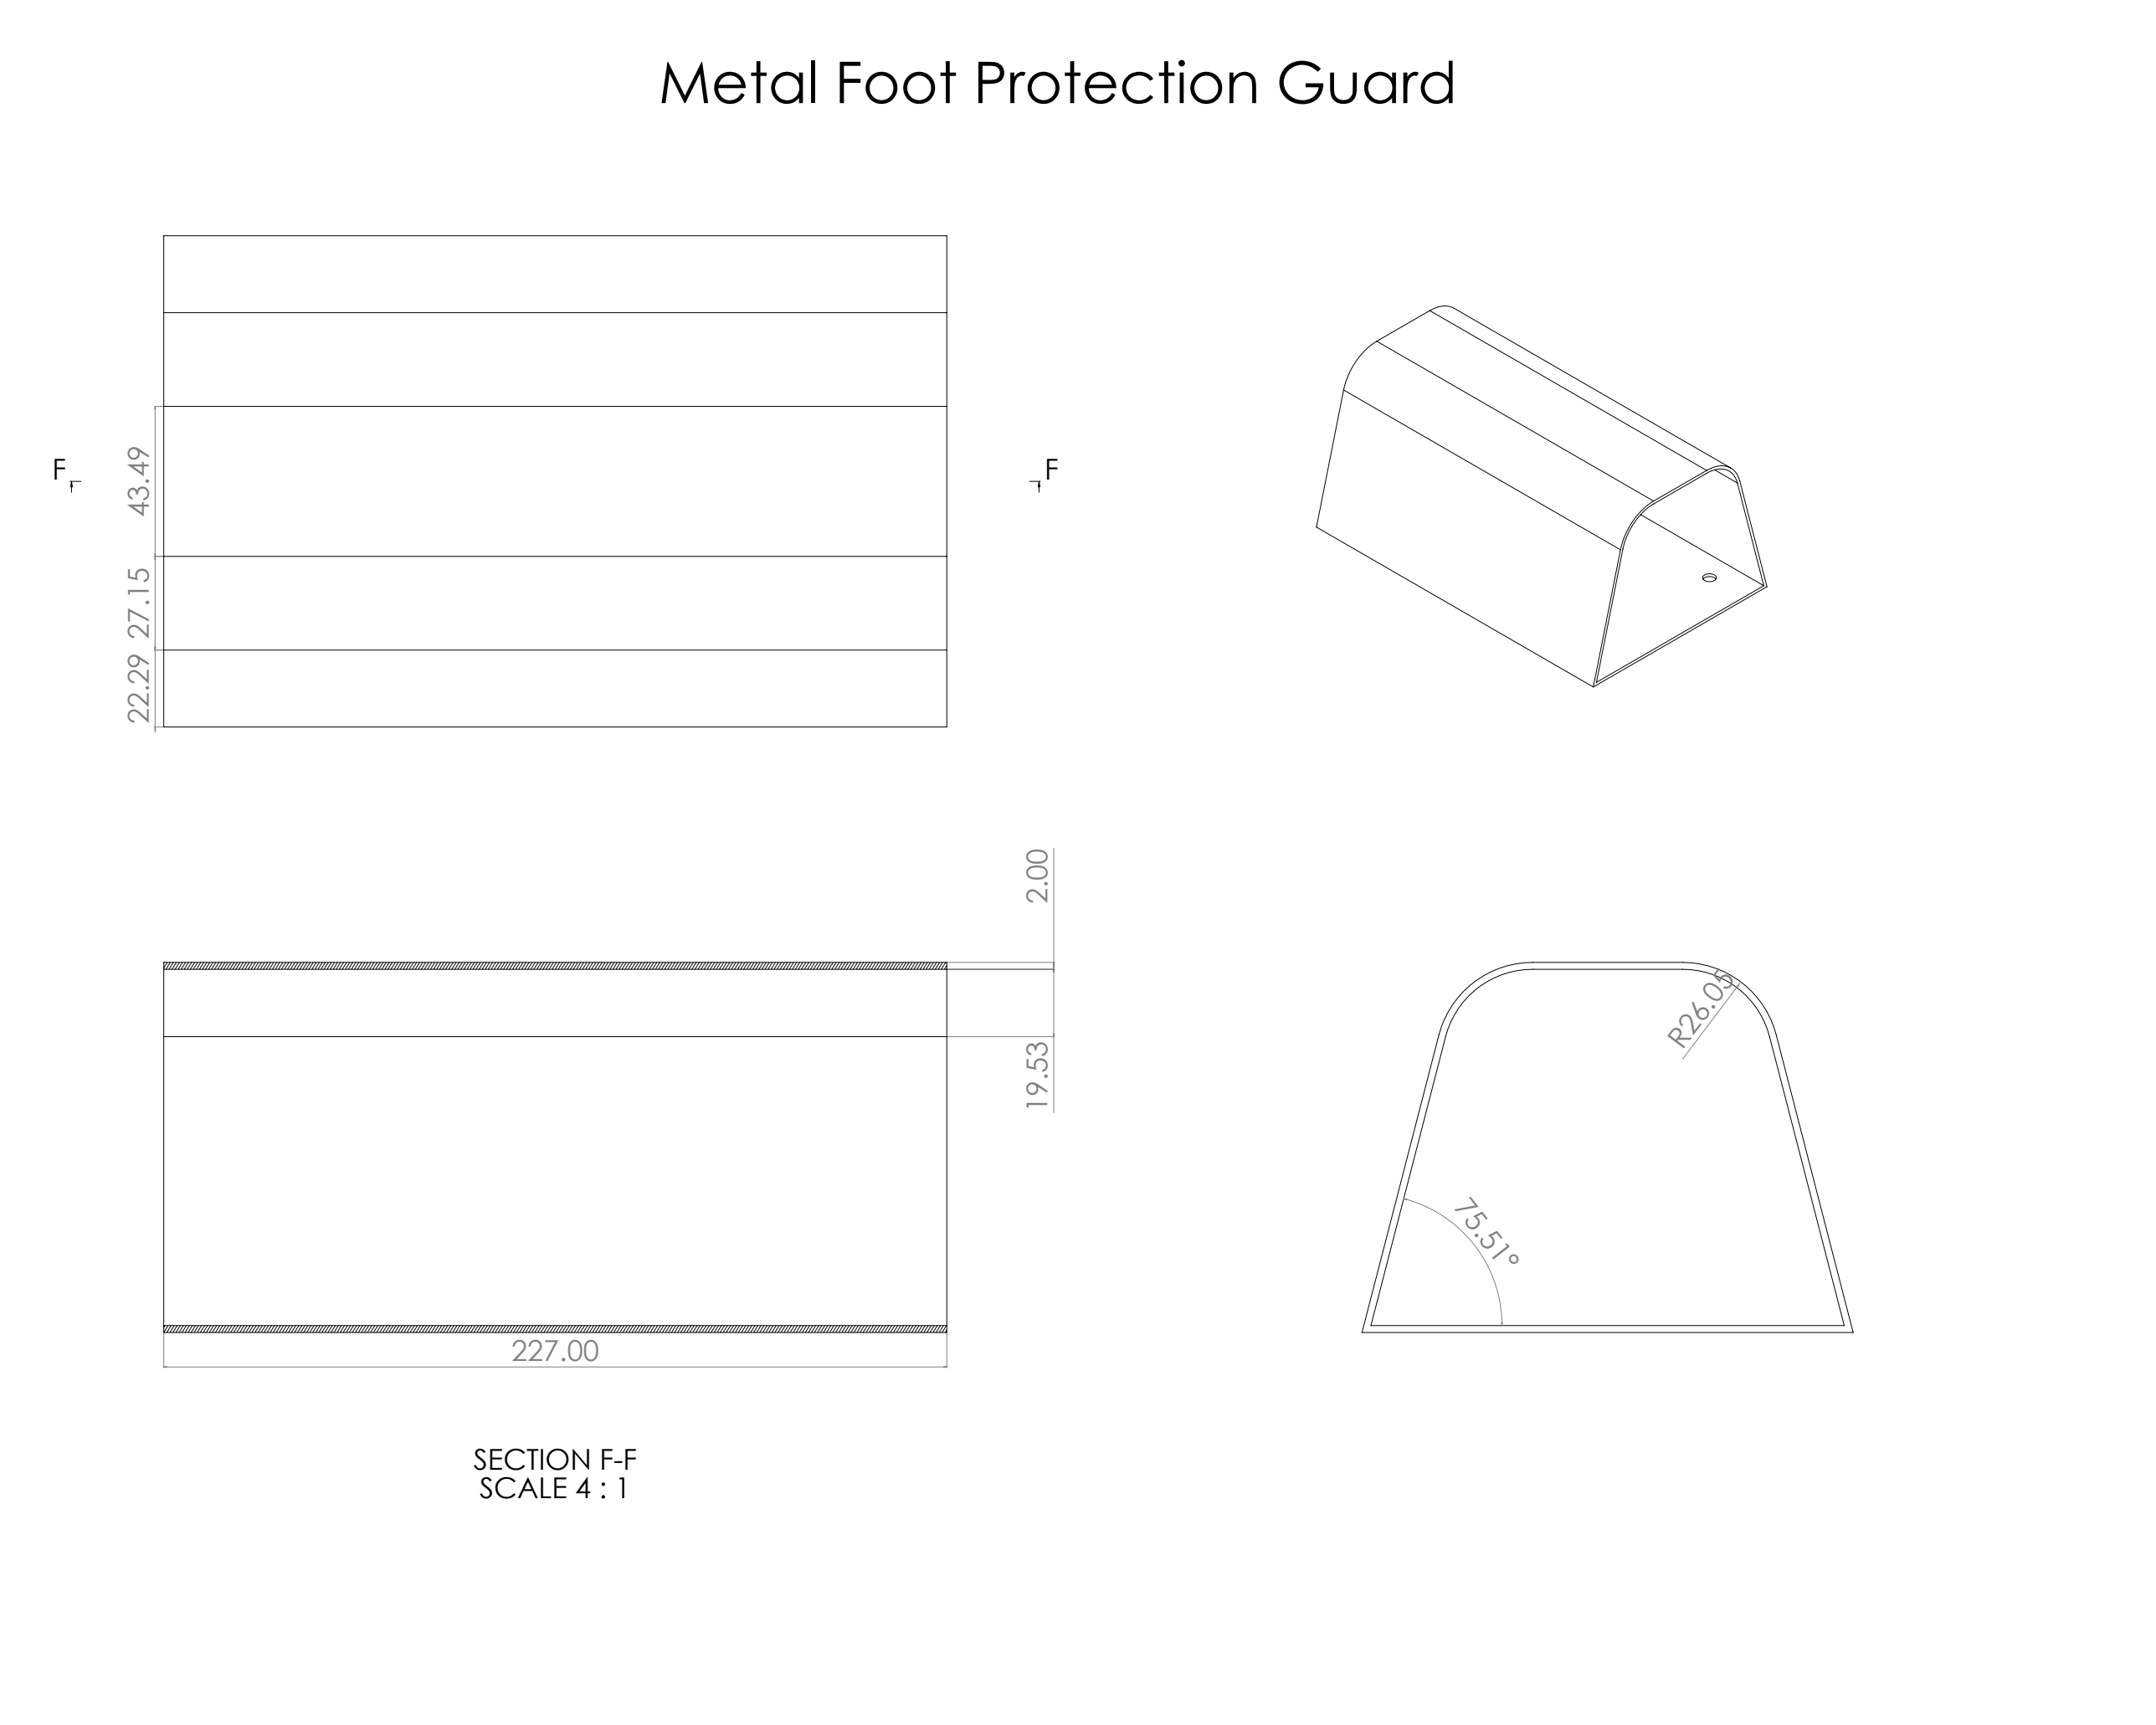
ISO-10303-21;
HEADER;
FILE_DESCRIPTION (('STEP AP214'),
    '1' );
FILE_NAME ('Metal Foot Protection Guard.step',
    '2026-10-25T20:52:49',
    ( '' ),
    ( '' ),
    'SwSTEP 2.0',
    'SolidWorks 2025',
    '' );
FILE_SCHEMA (( 'AUTOMOTIVE_DESIGN' ));
ENDSEC;

DATA;
#6=DIRECTION ( 'NONE',  ( 0.000000000000000000, 1.000000000000000000, 0.000000000000000000 ) ) ;
#417=ORIENTED_EDGE ( 'NONE', *, *, #24378, .F. ) ;
#442=ORIENTED_EDGE ( 'NONE', *, *, #84617, .T. ) ;
#778=VECTOR ( 'NONE', #36386, 1000.000000000000000 ) ;
#1124=ORIENTED_EDGE ( 'NONE', *, *, #88943, .T. ) ;
#1238=PLANE ( 'NONE',  #55318 ) ;
#1278=CARTESIAN_POINT ( 'NONE',  ( -113.5000000000000568, -218.8335761803644743, -447.4016117689005796 ) ) ;
#1316=LINE ( 'NONE', #58628, #74329 ) ;
#1432=CYLINDRICAL_SURFACE ( 'NONE', #55768, 26.04691768583017364 ) ;
#1539=DIRECTION ( 'NONE',  ( -1.000000000000000000, -0.000000000000000000, -0.000000000000000000 ) ) ;
#1792=LINE ( 'NONE', #80865, #778 ) ;
#1878=ORIENTED_EDGE ( 'NONE', *, *, #16109, .T. ) ;
#1900=DIRECTION ( 'NONE',  ( -1.000000000000000000, -0.000000000000000000, -0.000000000000000000 ) ) ;
#1936=ORIENTED_EDGE ( 'NONE', *, *, #63556, .T. ) ;
#1958=PRODUCT ( 'Metal Foot Protection Guard', 'Metal Foot Protection Guard', '', ( #38817 ) ) ;
#2011=AXIS2_PLACEMENT_3D ( 'NONE', #16154, #66807, #89023 ) ;
#2249=LINE ( 'NONE', #31133, #23268 ) ;
#2276=VERTEX_POINT ( 'NONE', #93668 ) ;
#2307=ORIENTED_EDGE ( 'NONE', *, *, #76975, .F. ) ;
#2323=VECTOR ( 'NONE', #62128, 1000.000000000000114 ) ;
#2326=DIRECTION ( 'NONE',  ( 0.000000000000000000, 1.000000000000000000, 0.000000000000000000 ) ) ;
#2997=CARTESIAN_POINT ( 'NONE',  ( -83.63170945779077670, -296.0521521680024080, -417.1172536214571096 ) ) ;
#3014=DIRECTION ( 'NONE',  ( 0.000000000000000000, 0.000000000000000000, 1.000000000000000000 ) ) ;
#3055=CARTESIAN_POINT ( 'NONE',  ( 113.5000000000000568, -218.8335761803644743, -490.8867980474134356 ) ) ;
#3161=ORIENTED_EDGE ( 'NONE', *, *, #12809, .F. ) ;
#3235=EDGE_CURVE ( 'NONE', #62642, #12065, #46260, .T. ) ;
#3595=AXIS2_PLACEMENT_3D ( 'NONE', #45296, #24471, #37283 ) ;
#3602=LINE ( 'NONE', #11632, #79019 ) ;
#3637=AXIS2_PLACEMENT_3D ( 'NONE', #49476, #63245, #84503 ) ;
#3779=ADVANCED_FACE ( 'NONE', ( #26838 ), #85054, .T. ) ;
#4574=UNCERTAINTY_MEASURE_WITH_UNIT (LENGTH_MEASURE( 1.000000000000000082E-05 ), #34987, 'distance_accuracy_value', 'NONE');
#4833=EDGE_CURVE ( 'NONE', #43507, #93231, #73286, .T. ) ;
#4839=ORIENTED_EDGE ( 'NONE', *, *, #80738, .T. ) ;
#4990=AXIS2_PLACEMENT_3D ( 'NONE', #56009, #66271, #51112 ) ;
#5017=CIRCLE ( 'NONE', #18666, 4.000000000000003553 ) ;
#5158=ORIENTED_EDGE ( 'NONE', *, *, #48217, .F. ) ;
#5173=ORIENTED_EDGE ( 'NONE', *, *, #11459, .F. ) ;
#5210=ORIENTED_EDGE ( 'NONE', *, *, #44156, .F. ) ;
#5394=ORIENTED_EDGE ( 'NONE', *, *, #33276, .T. ) ;
#5925=DIRECTION ( 'NONE',  ( 0.000000000000000000, 0.000000000000000000, 1.000000000000000000 ) ) ;
#6052=PLANE ( 'NONE',  #74600 ) ;
#6401=DIRECTION ( 'NONE',  ( 0.000000000000000000, -0.2502735790305607444, 0.9681751575201843485 ) ) ;
#6492=VECTOR ( 'NONE', #33731, 1000.000000000000000 ) ;
#6796=ORIENTED_EDGE ( 'NONE', *, *, #27340, .T. ) ;
#6987=FACE_BOUND ( 'NONE', #78000, .T. ) ;
#7172=( LENGTH_UNIT ( ) NAMED_UNIT ( * ) SI_UNIT ( .MILLI., .METRE. ) );
#7304=EDGE_LOOP ( 'NONE', ( #59580, #39641, #11949, #25899 ) ) ;
#7427=VECTOR ( 'NONE', #91516, 1000.000000000000000 ) ;
#7537=CARTESIAN_POINT ( 'NONE',  ( 113.5000000000000568, -296.0521521680024080, -400.5374811273811702 ) ) ;
#7762=PRODUCT_DEFINITION_CONTEXT ( 'detailed design', #78364, 'design' ) ;
#8035=VECTOR ( 'NONE', #18647, 1000.000000000000000 ) ;
#8052=AXIS2_PLACEMENT_3D ( 'NONE', #67191, #2326, #31206 ) ;
#8263=VECTOR ( 'NONE', #42060, 1000.000000000000000 ) ;
#8490=CARTESIAN_POINT ( 'NONE',  ( 113.5000000000000568, -296.0521521680024080, -537.7509286889328450 ) ) ;
#8572=ADVANCED_FACE ( 'NONE', ( #49622 ), #42507, .F. ) ;
#8832=VECTOR ( 'NONE', #60146, 1000.000000000000000 ) ;
#9134=DIRECTION ( 'NONE',  ( 0.000000000000000000, 0.000000000000000000, 1.000000000000000000 ) ) ;
#9174=CARTESIAN_POINT ( 'NONE',  ( -83.63170945779074827, -298.0521521680024080, -525.1711561948568487 ) ) ;
#9287=DIRECTION ( 'NONE',  ( 0.000000000000000000, 0.000000000000000000, 1.000000000000000000 ) ) ;
#9340=CARTESIAN_POINT ( 'NONE',  ( -113.5000000000000568, -298.0521521680024080, -397.9547385950631337 ) ) ;
#9353=EDGE_CURVE ( 'NONE', #42812, #91222, #48447, .T. ) ;
#9407=LINE ( 'NONE', #9886, #56602 ) ;
#9526=CIRCLE ( 'NONE', #18677, 4.000000000000003553 ) ;
#9540=ORIENTED_EDGE ( 'NONE', *, *, #63681, .T. ) ;
#9616=VERTEX_POINT ( 'NONE', #11064 ) ;
#9664=VECTOR ( 'NONE', #74863, 1000.000000000000000 ) ;
#9758=LINE ( 'NONE', #89272, #23223 ) ;
#9886=CARTESIAN_POINT ( 'NONE',  ( -83.63170945779074827, -373.0521521680024648, -517.1711561948568487 ) ) ;
#10053=CARTESIAN_POINT ( 'NONE',  ( -113.5000000000000568, -296.0521521680024080, -400.5374811273811702 ) ) ;
#10064=DIRECTION ( 'NONE',  ( 0.000000000000000000, 0.000000000000000000, -1.000000000000000000 ) ) ;
#10078=ORIENTED_EDGE ( 'NONE', *, *, #83711, .T. ) ;
#10254=VERTEX_POINT ( 'NONE', #23518 ) ;
#10301=DIRECTION ( 'NONE',  ( -1.000000000000000000, -0.000000000000000000, -0.000000000000000000 ) ) ;
#10703=CARTESIAN_POINT ( 'NONE',  ( -113.5000000000000568, -212.3147208684173677, -516.1047766808072765 ) ) ;
#10768=DIRECTION ( 'NONE',  ( 0.000000000000000000, 1.000000000000000000, -0.000000000000000000 ) ) ;
#11004=CARTESIAN_POINT ( 'NONE',  ( -113.5000000000000568, -192.7866584945343504, -447.4016117689005796 ) ) ;
#11062=ORIENTED_EDGE ( 'NONE', *, *, #17386, .T. ) ;
#11064=CARTESIAN_POINT ( 'NONE',  ( -83.63170945779077670, -296.0521521680024080, -421.1172536214571096 ) ) ;
#11141=VECTOR ( 'NONE', #68705, 1000.000000000000000 ) ;
#11159=CIRCLE ( 'NONE', #3595, 4.000000000000003553 ) ;
#11217=VECTOR ( 'NONE', #42131, 1000.000000000000000 ) ;
#11220=AXIS2_PLACEMENT_3D ( 'NONE', #68307, #26618, #10064 ) ;
#11228=CIRCLE ( 'NONE', #12737, 4.000000000000003553 ) ;
#11384=CARTESIAN_POINT ( 'NONE',  ( 85.55100297371598117, -373.0521521680024648, -417.1172536214571096 ) ) ;
#11459=EDGE_CURVE ( 'NONE', #56922, #42812, #78843, .T. ) ;
#11572=ORIENTED_EDGE ( 'NONE', *, *, #57340, .F. ) ;
#11597=ADVANCED_FACE ( 'NONE', ( #34821 ), #92559, .F. ) ;
#11632=CARTESIAN_POINT ( 'NONE',  ( 113.5000000000000568, -192.7866584945343504, -490.8867980474134356 ) ) ;
#11690=LINE ( 'NONE', #31611, #47780 ) ;
#11793=VERTEX_POINT ( 'NONE', #9174 ) ;
#11949=ORIENTED_EDGE ( 'NONE', *, *, #24378, .T. ) ;
#11985=FACE_OUTER_BOUND ( 'NONE', #85658, .T. ) ;
#12065=VERTEX_POINT ( 'NONE', #81159 ) ;
#12119=DIRECTION ( 'NONE',  ( 0.000000000000000000, 0.000000000000000000, 1.000000000000000000 ) ) ;
#12292=AXIS2_PLACEMENT_3D ( 'NONE', #39594, #90715, #47174 ) ;
#12596=DIRECTION ( 'NONE',  ( 0.000000000000000000, 0.000000000000000000, 1.000000000000000000 ) ) ;
#12668=VECTOR ( 'NONE', #72103, 1000.000000000000000 ) ;
#12724=AXIS2_PLACEMENT_3D ( 'NONE', #43548, #6, #35985 ) ;
#12737=AXIS2_PLACEMENT_3D ( 'NONE', #90881, #26997, #70096 ) ;
#12809=EDGE_CURVE ( 'NONE', #47975, #62368, #77199, .T. ) ;
#13122=DIRECTION ( 'NONE',  ( 0.000000000000000000, 0.000000000000000000, 1.000000000000000000 ) ) ;
#13127=ORIENTED_EDGE ( 'NONE', *, *, #73397, .F. ) ;
#13224=LINE ( 'NONE', #63892, #8263 ) ;
#13625=EDGE_CURVE ( 'NONE', #81684, #49342, #44460, .T. ) ;
#13690=CARTESIAN_POINT ( 'NONE',  ( -113.5000000000000568, -296.0521521680024080, -537.7509286889328450 ) ) ;
#13868=EDGE_CURVE ( 'NONE', #10254, #49342, #9407, .T. ) ;
#14078=ORIENTED_EDGE ( 'NONE', *, *, #37019, .F. ) ;
#14096=FACE_OUTER_BOUND ( 'NONE', #76110, .T. ) ;
#14616=FACE_BOUND ( 'NONE', #27456, .T. ) ;
#14990=DIRECTION ( 'NONE',  ( -1.000000000000000000, -0.000000000000000000, -0.000000000000000000 ) ) ;
#15544=VECTOR ( 'NONE', #14990, 1000.000000000000000 ) ;
#15625=EDGE_LOOP ( 'NONE', ( #53579, #46500, #71098, #20534 ) ) ;
#15643=FACE_OUTER_BOUND ( 'NONE', #7304, .T. ) ;
#15682=VECTOR ( 'NONE', #78384, 1000.000000000000000 ) ;
#15729=CARTESIAN_POINT ( 'NONE',  ( 113.5000000000000568, -218.8335761803644743, -490.8867980474134356 ) ) ;
#16109=EDGE_CURVE ( 'NONE', #36642, #59451, #59215, .T. ) ;
#16152=ORIENTED_EDGE ( 'NONE', *, *, #87773, .F. ) ;
#16154=CARTESIAN_POINT ( 'NONE',  ( 113.5000000000000568, -298.0521521680024080, -397.9547385950631337 ) ) ;
#16280=DIRECTION ( 'NONE',  ( 0.000000000000000000, 1.000000000000000000, -0.000000000000000000 ) ) ;
#16610=VERTEX_POINT ( 'NONE', #17359 ) ;
#16751=CARTESIAN_POINT ( 'NONE',  ( 85.55100297371598117, -298.0521521680024080, -413.1172536214571096 ) ) ;
#17028=EDGE_CURVE ( 'NONE', #11793, #10254, #78948, .T. ) ;
#17038=PLANE ( 'NONE',  #56694 ) ;
#17200=CYLINDRICAL_SURFACE ( 'NONE', #59412, 4.000000000000003553 ) ;
#17359=CARTESIAN_POINT ( 'NONE',  ( 85.55100297371609486, -296.0521521680024080, -517.1711561948568487 ) ) ;
#17386=EDGE_CURVE ( 'NONE', #83022, #62368, #77460, .T. ) ;
#17968=DIRECTION ( 'NONE',  ( 0.000000000000000000, -0.9681751575201845705, -0.2502735790305594121 ) ) ;
#18379=AXIS2_PLACEMENT_3D ( 'NONE', #1278, #36796, #9287 ) ;
#18420=ORIENTED_EDGE ( 'NONE', *, *, #41482, .F. ) ;
#18451=EDGE_LOOP ( 'NONE', ( #81543, #43240, #57627, #38795 ) ) ;
#18490=CARTESIAN_POINT ( 'NONE',  ( 85.55100297371598117, -373.0521521680024648, -421.1172536214571096 ) ) ;
#18518=ORIENTED_EDGE ( 'NONE', *, *, #62083, .T. ) ;
#18585=ORIENTED_EDGE ( 'NONE', *, *, #17028, .F. ) ;
#18647=DIRECTION ( 'NONE',  ( 0.000000000000000000, 0.000000000000000000, -1.000000000000000000 ) ) ;
#18666=AXIS2_PLACEMENT_3D ( 'NONE', #60916, #53801, #89762 ) ;
#18677=AXIS2_PLACEMENT_3D ( 'NONE', #58278, #92351, #27995 ) ;
#18940=AXIS2_PLACEMENT_3D ( 'NONE', #90959, #40773, #33703 ) ;
#18980=LINE ( 'NONE', #83344, #11141 ) ;
#19066=LINE ( 'NONE', #54562, #47269 ) ;
#19232=PRODUCT_DEFINITION ( 'UNKNOWN', '', #50708, #7762 ) ;
#19258=ORIENTED_EDGE ( 'NONE', *, *, #88840, .T. ) ;
#19434=CARTESIAN_POINT ( 'NONE',  ( 113.5000000000000568, -190.7866584945343220, -490.8867980474134356 ) ) ;
#19749=LINE ( 'NONE', #49566, #47581 ) ;
#19761=EDGE_LOOP ( 'NONE', ( #31495, #72178, #26521, #82940 ) ) ;
#19828=ORIENTED_EDGE ( 'NONE', *, *, #17386, .F. ) ;
#19877=ORIENTED_EDGE ( 'NONE', *, *, #47034, .T. ) ;
#20150=EDGE_CURVE ( 'NONE', #62642, #36954, #86465, .T. ) ;
#20278=CIRCLE ( 'NONE', #3637, 4.000000000000003553 ) ;
#20299=ORIENTED_EDGE ( 'NONE', *, *, #63681, .F. ) ;
#20534=ORIENTED_EDGE ( 'NONE', *, *, #20150, .T. ) ;
#20637=DIRECTION ( 'NONE',  ( 0.000000000000000000, 0.000000000000000000, 1.000000000000000000 ) ) ;
#21150=ORIENTED_EDGE ( 'NONE', *, *, #37532, .F. ) ;
#21204=ADVANCED_FACE ( 'NONE', ( #39998 ), #34334, .F. ) ;
#21313=CARTESIAN_POINT ( 'NONE',  ( 113.5000000000000568, -211.8141737103562434, -420.2472828204663529 ) ) ;
#21449=ORIENTED_EDGE ( 'NONE', *, *, #40622, .F. ) ;
#21618=CIRCLE ( 'NONE', #66969, 26.04691768583017364 ) ;
#22565=DIRECTION ( 'NONE',  ( 0.000000000000000000, 0.9681751575201842375, 0.2502735790305606889 ) ) ;
#22793=EDGE_CURVE ( 'NONE', #29874, #9616, #86552, .T. ) ;
#22928=LINE ( 'NONE', #23410, #36160 ) ;
#23184=VECTOR ( 'NONE', #47355, 1000.000000000000000 ) ;
#23194=CARTESIAN_POINT ( 'NONE',  ( -83.63170945779074827, -296.0521521680024080, -525.1711561948568487 ) ) ;
#23223=VECTOR ( 'NONE', #22565, 1000.000000000000114 ) ;
#23268=VECTOR ( 'NONE', #60019, 1000.000000000000114 ) ;
#23410=CARTESIAN_POINT ( 'NONE',  ( 113.5000000000000568, -298.0521521680024080, -397.9547385950631337 ) ) ;
#23518=CARTESIAN_POINT ( 'NONE',  ( -83.63170945779074827, -298.0521521680024080, -517.1711561948568487 ) ) ;
#24130=FACE_BOUND ( 'NONE', #61458, .T. ) ;
#24202=CARTESIAN_POINT ( 'NONE',  ( 113.5000000000000568, -192.7866584945343504, -447.4016117689005796 ) ) ;
#24218=ORIENTED_EDGE ( 'NONE', *, *, #20150, .F. ) ;
#24378=EDGE_CURVE ( 'NONE', #59329, #45702, #21618, .T. ) ;
#24471=DIRECTION ( 'NONE',  ( 0.000000000000000000, 1.000000000000000000, -0.000000000000000000 ) ) ;
#24482=CYLINDRICAL_SURFACE ( 'NONE', #12292, 4.000000000000003553 ) ;
#24501=ADVANCED_FACE ( 'NONE', ( #49483 ), #42361, .T. ) ;
#24656=CARTESIAN_POINT ( 'NONE',  ( 113.5000000000000568, -190.7866584945343504, -447.4016117689005796 ) ) ;
#24719=AXIS2_PLACEMENT_3D ( 'NONE', #52941, #58675, #80428 ) ;
#24795=AXIS2_PLACEMENT_3D ( 'NONE', #83095, #46641, #61365 ) ;
#24966=VERTEX_POINT ( 'NONE', #16751 ) ;
#24977=DIRECTION ( 'NONE',  ( 0.000000000000000000, 0.9681751575201845705, 0.2502735790305594676 ) ) ;
#25097=EDGE_CURVE ( 'NONE', #36396, #62468, #29192, .T. ) ;
#25137=DIRECTION ( 'NONE',  ( -1.000000000000000000, -0.000000000000000000, -0.000000000000000000 ) ) ;
#25427=CARTESIAN_POINT ( 'NONE',  ( -83.63170945779077670, -298.0521521680024080, -421.1172536214571096 ) ) ;
#25499=CARTESIAN_POINT ( 'NONE',  ( -83.63170945779077670, -298.0521521680024080, -417.1172536214571096 ) ) ;
#25663=VECTOR ( 'NONE', #69750, 1000.000000000000000 ) ;
#25825=CARTESIAN_POINT ( 'NONE',  ( 85.55100297371609486, -373.0521521680024648, -517.1711561948568487 ) ) ;
#25899=ORIENTED_EDGE ( 'NONE', *, *, #27474, .T. ) ;
#25906=ADVANCED_FACE ( 'NONE', ( #63142 ), #92435, .F. ) ;
#25988=CARTESIAN_POINT ( 'NONE',  ( -113.5000000000000568, -211.8141737103562434, -420.2472828204663529 ) ) ;
#26374=AXIS2_PLACEMENT_3D ( 'NONE', #11384, #55885, #77662 ) ;
#26406=CARTESIAN_POINT ( 'NONE',  ( -83.63170945779077670, -296.0521521680024080, -413.1172536214571096 ) ) ;
#26521=ORIENTED_EDGE ( 'NONE', *, *, #92612, .F. ) ;
#26576=STYLED_ITEM('',(#93745),#91220);
#26618=DIRECTION ( 'NONE',  ( 1.000000000000000000, 0.000000000000000000, 0.000000000000000000 ) ) ;
#26725=VERTEX_POINT ( 'NONE', #31215 ) ;
#26753=ORIENTED_EDGE ( 'NONE', *, *, #54874, .F. ) ;
#26784=LINE ( 'NONE', #69395, #69956 ) ;
#26790=DIRECTION ( 'NONE',  ( 0.000000000000000000, 0.000000000000000000, -1.000000000000000000 ) ) ;
#26838=FACE_OUTER_BOUND ( 'NONE', #29382, .T. ) ;
#26936=DIRECTION ( 'NONE',  ( -0.000000000000000000, 1.000000000000000000, 0.000000000000000000 ) ) ;
#26993=EDGE_CURVE ( 'NONE', #62368, #42343, #66156, .T. ) ;
#26997=DIRECTION ( 'NONE',  ( -0.000000000000000000, 1.000000000000000000, 0.000000000000000000 ) ) ;
#27340=EDGE_CURVE ( 'NONE', #86290, #16610, #41184, .T. ) ;
#27456=EDGE_LOOP ( 'NONE', ( #13127, #57449 ) ) ;
#27474=EDGE_CURVE ( 'NONE', #45702, #59451, #26784, .T. ) ;
#27503=EDGE_CURVE ( 'NONE', #32344, #93231, #3602, .T. ) ;
#27715=DIRECTION ( 'NONE',  ( 1.000000000000000000, 0.000000000000000000, -0.000000000000000000 ) ) ;
#27811=AXIS2_PLACEMENT_3D ( 'NONE', #92152, #71340, #13122 ) ;
#27995=DIRECTION ( 'NONE',  ( 0.000000000000000000, 0.000000000000000000, 1.000000000000000000 ) ) ;
#28110=ORIENTED_EDGE ( 'NONE', *, *, #46184, .T. ) ;
#28339=VERTEX_POINT ( 'NONE', #72116 ) ;
#28547=DIRECTION ( 'NONE',  ( 1.000000000000000000, 0.000000000000000000, 0.000000000000000000 ) ) ;
#28573=ORIENTED_EDGE ( 'NONE', *, *, #84617, .F. ) ;
#28694=ADVANCED_FACE ( 'NONE', ( #38416 ), #89059, .T. ) ;
#28804=CIRCLE ( 'NONE', #43914, 4.000000000000003553 ) ;
#28860=ORIENTED_EDGE ( 'NONE', *, *, #92612, .T. ) ;
#29034=LINE ( 'NONE', #65051, #79325 ) ;
#29126=VECTOR ( 'NONE', #88842, 1000.000000000000000 ) ;
#29188=CARTESIAN_POINT ( 'NONE',  ( -113.5000000000000568, -218.8335761803644743, -447.4016117689005796 ) ) ;
#29192=CIRCLE ( 'NONE', #42837, 4.000000000000003553 ) ;
#29382=EDGE_LOOP ( 'NONE', ( #47639, #21150, #5210, #41236 ) ) ;
#29514=CLOSED_SHELL ( 'NONE', ( #63024, #58384, #8572, #25906, #86201, #90366, #64306, #71705, #86978, #28694, #11597, #3779, #45814, #65404, #57136, #24501, #56322, #67787, #21204, #57559, #74931, #33563 ) ) ;
#29531=ORIENTED_EDGE ( 'NONE', *, *, #72303, .F. ) ;
#29874=VERTEX_POINT ( 'NONE', #26406 ) ;
#30154=DIRECTION ( 'NONE',  ( -0.000000000000000000, -0.000000000000000000, 1.000000000000000000 ) ) ;
#30209=CARTESIAN_POINT ( 'NONE',  ( -83.63170945779077670, -373.0521521680024648, -421.1172536214571096 ) ) ;
#30870=DIRECTION ( 'NONE',  ( -1.000000000000000000, -0.000000000000000000, -0.000000000000000000 ) ) ;
#30965=DIRECTION ( 'NONE',  ( 0.000000000000000000, 0.000000000000000000, -1.000000000000000000 ) ) ;
#31133=CARTESIAN_POINT ( 'NONE',  ( 113.5000000000000568, -296.0521521680024080, -400.5374811273811702 ) ) ;
#31206=DIRECTION ( 'NONE',  ( 0.000000000000000000, 0.000000000000000000, 1.000000000000000000 ) ) ;
#31215=CARTESIAN_POINT ( 'NONE',  ( -113.5000000000000568, -298.0521521680024080, -397.9547385950631337 ) ) ;
#31299=FACE_OUTER_BOUND ( 'NONE', #48421, .T. ) ;
#31495=ORIENTED_EDGE ( 'NONE', *, *, #26993, .T. ) ;
#31611=CARTESIAN_POINT ( 'NONE',  ( 85.55100297371598117, -373.0521521680024648, -413.1172536214571096 ) ) ;
#32008=CARTESIAN_POINT ( 'NONE',  ( -113.5000000000000568, -190.7866584945343504, -447.4016117689005796 ) ) ;
#32177=FACE_OUTER_BOUND ( 'NONE', #62147, .T. ) ;
#32191=VERTEX_POINT ( 'NONE', #48875 ) ;
#32344=VERTEX_POINT ( 'NONE', #73466 ) ;
#32571=DIRECTION ( 'NONE',  ( 1.000000000000000000, 0.000000000000000000, -0.000000000000000000 ) ) ;
#32846=EDGE_CURVE ( 'NONE', #33034, #42343, #75779, .T. ) ;
#33034=VERTEX_POINT ( 'NONE', #52591 ) ;
#33131=ORIENTED_EDGE ( 'NONE', *, *, #88943, .F. ) ;
#33276=EDGE_CURVE ( 'NONE', #24966, #2276, #11228, .T. ) ;
#33562=PLANE ( 'NONE',  #73301 ) ;
#33563=ADVANCED_FACE ( 'NONE', ( #33622 ), #77187, .F. ) ;
#33622=FACE_OUTER_BOUND ( 'NONE', #60401, .T. ) ;
#33703=DIRECTION ( 'NONE',  ( 1.000000000000000000, 0.000000000000000000, 0.000000000000000000 ) ) ;
#33731=DIRECTION ( 'NONE',  ( -0.000000000000000000, -0.000000000000000000, 1.000000000000000000 ) ) ;
#33765=LINE ( 'NONE', #40831, #25663 ) ;
#33970=CARTESIAN_POINT ( 'NONE',  ( 85.55100297371598117, -296.0521521680024080, -421.1172536214571096 ) ) ;
#34334=CYLINDRICAL_SURFACE ( 'NONE', #42697, 4.000000000000003553 ) ;
#34351=EDGE_CURVE ( 'NONE', #62468, #36396, #38245, .T. ) ;
#34433=EDGE_LOOP ( 'NONE', ( #5394, #4839 ) ) ;
#34821=FACE_OUTER_BOUND ( 'NONE', #19761, .T. ) ;
#34974=ORIENTED_EDGE ( 'NONE', *, *, #93458, .F. ) ;
#34975=FACE_BOUND ( 'NONE', #60847, .T. ) ;
#34987=( LENGTH_UNIT ( ) NAMED_UNIT ( * ) SI_UNIT ( .MILLI., .METRE. ) );
#35165=CARTESIAN_POINT ( 'NONE',  ( -83.63170945779077670, -373.0521521680024648, -417.1172536214571096 ) ) ;
#35273=DIRECTION ( 'NONE',  ( 0.000000000000000000, -0.9681751575201842375, -0.2502735790305606889 ) ) ;
#35461=ORIENTED_EDGE ( 'NONE', *, *, #65933, .F. ) ;
#35632=EDGE_CURVE ( 'NONE', #28339, #43507, #57427, .T. ) ;
#35763=CARTESIAN_POINT ( 'NONE',  ( 113.5000000000000568, -296.0521521680024080, -400.5374811273811702 ) ) ;
#35912=CARTESIAN_POINT ( 'NONE',  ( 113.5000000000000568, -296.0521521680024080, -400.5374811273811702 ) ) ;
#35985=DIRECTION ( 'NONE',  ( 0.000000000000000000, 0.000000000000000000, 1.000000000000000000 ) ) ;
#36137=CYLINDRICAL_SURFACE ( 'NONE', #86365, 26.04691768583011680 ) ;
#36160=VECTOR ( 'NONE', #53688, 1000.000000000000227 ) ;
#36209=DIRECTION ( 'NONE',  ( 0.000000000000000000, 1.000000000000000000, 0.000000000000000000 ) ) ;
#36285=DIRECTION ( 'NONE',  ( 0.000000000000000000, 0.000000000000000000, 1.000000000000000000 ) ) ;
#36386=DIRECTION ( 'NONE',  ( -0.000000000000000000, -0.000000000000000000, 1.000000000000000000 ) ) ;
#36396=VERTEX_POINT ( 'NONE', #52151 ) ;
#36491=AXIS2_PLACEMENT_3D ( 'NONE', #64374, #26936, #71921 ) ;
#36642=VERTEX_POINT ( 'NONE', #84286 ) ;
#36796=DIRECTION ( 'NONE',  ( 1.000000000000000000, 0.000000000000000000, -0.000000000000000000 ) ) ;
#36806=EDGE_CURVE ( 'NONE', #26725, #36954, #18980, .T. ) ;
#36954=VERTEX_POINT ( 'NONE', #85241 ) ;
#37019=EDGE_CURVE ( 'NONE', #2276, #62468, #76734, .T. ) ;
#37283=DIRECTION ( 'NONE',  ( 0.000000000000000000, 0.000000000000000000, -1.000000000000000000 ) ) ;
#37511=CARTESIAN_POINT ( 'NONE',  ( 113.5000000000000568, -218.8335761803644743, -490.8867980474134356 ) ) ;
#37532=EDGE_CURVE ( 'NONE', #74793, #87260, #79554, .T. ) ;
#37881=CIRCLE ( 'NONE', #87766, 26.04691768583011680 ) ;
#37901=ORIENTED_EDGE ( 'NONE', *, *, #35632, .F. ) ;
#37982=VERTEX_POINT ( 'NONE', #8490 ) ;
#38014=EDGE_LOOP ( 'NONE', ( #63002, #21449, #51278, #67111 ) ) ;
#38221=AXIS2_PLACEMENT_3D ( 'NONE', #2997, #16280, #30965 ) ;
#38245=CIRCLE ( 'NONE', #56468, 4.000000000000003553 ) ;
#38416=FACE_OUTER_BOUND ( 'NONE', #42687, .T. ) ;
#38490=ORIENTED_EDGE ( 'NONE', *, *, #13625, .T. ) ;
#38526=DIRECTION ( 'NONE',  ( 0.000000000000000000, 0.000000000000000000, -1.000000000000000000 ) ) ;
#38600=VECTOR ( 'NONE', #88428, 1000.000000000000000 ) ;
#38642=CARTESIAN_POINT ( 'NONE',  ( 85.55100297371609486, -296.0521521680024080, -521.1711561948568487 ) ) ;
#38727=VECTOR ( 'NONE', #83179, 1000.000000000000227 ) ;
#38795=ORIENTED_EDGE ( 'NONE', *, *, #92638, .F. ) ;
#38817=PRODUCT_CONTEXT ( 'NONE', #83158, 'mechanical' ) ;
#38918=ORIENTED_EDGE ( 'NONE', *, *, #74417, .T. ) ;
#38951=ORIENTED_EDGE ( 'NONE', *, *, #83939, .T. ) ;
#39107=CARTESIAN_POINT ( 'NONE',  ( 113.5000000000000568, -211.8141737103562434, -518.0411269958476623 ) ) ;
#39248=CARTESIAN_POINT ( 'NONE',  ( 85.55100297371609486, -296.0521521680024080, -525.1711561948568487 ) ) ;
#39473=DIRECTION ( 'NONE',  ( 1.000000000000000000, 0.000000000000000000, 0.000000000000000000 ) ) ;
#39594=CARTESIAN_POINT ( 'NONE',  ( -83.63170945779074827, -373.0521521680024648, -521.1711561948568487 ) ) ;
#39641=ORIENTED_EDGE ( 'NONE', *, *, #62083, .F. ) ;
#39844=VECTOR ( 'NONE', #24977, 1000.000000000000227 ) ;
#39966=EDGE_LOOP ( 'NONE', ( #20299, #71251, #1124, #18518 ) ) ;
#39998=FACE_OUTER_BOUND ( 'NONE', #69096, .T. ) ;
#40316=ORIENTED_EDGE ( 'NONE', *, *, #22793, .T. ) ;
#40452=DIRECTION ( 'NONE',  ( -0.000000000000000000, 1.000000000000000000, -0.000000000000000000 ) ) ;
#40514=ORIENTED_EDGE ( 'NONE', *, *, #50161, .F. ) ;
#40622=EDGE_CURVE ( 'NONE', #10254, #11793, #5017, .T. ) ;
#40773=DIRECTION ( 'NONE',  ( 0.000000000000000000, 0.000000000000000000, 1.000000000000000000 ) ) ;
#40831=CARTESIAN_POINT ( 'NONE',  ( -83.63170945779074827, -373.0521521680024648, -525.1711561948568487 ) ) ;
#40834=CARTESIAN_POINT ( 'NONE',  ( -83.63170945779077670, -373.0521521680024648, -417.1172536214571096 ) ) ;
#40952=DIRECTION ( 'NONE',  ( 0.000000000000000000, 0.000000000000000000, 1.000000000000000000 ) ) ;
#41184=CIRCLE ( 'NONE', #74465, 4.000000000000003553 ) ;
#41236=ORIENTED_EDGE ( 'NONE', *, *, #32846, .T. ) ;
#41482=EDGE_CURVE ( 'NONE', #16610, #86290, #77613, .T. ) ;
#41493=EDGE_LOOP ( 'NONE', ( #34974, #64302, #38951, #84428 ) ) ;
#41569=DIRECTION ( 'NONE',  ( -0.000000000000000000, 1.000000000000000000, -0.000000000000000000 ) ) ;
#41645=ORIENTED_EDGE ( 'NONE', *, *, #25097, .F. ) ;
#41963=ORIENTED_EDGE ( 'NONE', *, *, #87773, .T. ) ;
#42060=DIRECTION ( 'NONE',  ( -0.000000000000000000, 1.000000000000000000, -0.000000000000000000 ) ) ;
#42131=DIRECTION ( 'NONE',  ( -1.000000000000000000, -0.000000000000000000, -0.000000000000000000 ) ) ;
#42343=VERTEX_POINT ( 'NONE', #65231 ) ;
#42361=PLANE ( 'NONE',  #79083 ) ;
#42462=ORIENTED_EDGE ( 'NONE', *, *, #55666, .F. ) ;
#42507=CYLINDRICAL_SURFACE ( 'NONE', #80903, 4.000000000000003553 ) ;
#42530=FACE_BOUND ( 'NONE', #61996, .T. ) ;
#42580=FACE_OUTER_BOUND ( 'NONE', #41493, .T. ) ;
#42687=EDGE_LOOP ( 'NONE', ( #11062, #3161, #35461, #81507 ) ) ;
#42697=AXIS2_PLACEMENT_3D ( 'NONE', #91112, #40452, #5925 ) ;
#42812=VERTEX_POINT ( 'NONE', #69640 ) ;
#42837=AXIS2_PLACEMENT_3D ( 'NONE', #80681, #73595, #38526 ) ;
#42924=ORIENTED_EDGE ( 'NONE', *, *, #87369, .T. ) ;
#42989=VECTOR ( 'NONE', #25137, 1000.000000000000000 ) ;
#43156=ORIENTED_EDGE ( 'NONE', *, *, #3235, .T. ) ;
#43240=ORIENTED_EDGE ( 'NONE', *, *, #37019, .T. ) ;
#43507=VERTEX_POINT ( 'NONE', #10703 ) ;
#43548=CARTESIAN_POINT ( 'NONE',  ( -83.63170945779074827, -296.0521521680024080, -521.1711561948568487 ) ) ;
#43838=ORIENTED_EDGE ( 'NONE', *, *, #27340, .F. ) ;
#43914=AXIS2_PLACEMENT_3D ( 'NONE', #78396, #49040, #12596 ) ;
#44156=EDGE_CURVE ( 'NONE', #33034, #74793, #64793, .T. ) ;
#44313=CIRCLE ( 'NONE', #24719, 28.04691768583012035 ) ;
#44460=CIRCLE ( 'NONE', #12724, 4.000000000000003553 ) ;
#44508=EDGE_LOOP ( 'NONE', ( #64959, #82454 ) ) ;
#44513=CARTESIAN_POINT ( 'NONE',  ( 113.5000000000000568, -218.8335761803644743, -447.4016117689005796 ) ) ;
#45296=CARTESIAN_POINT ( 'NONE',  ( -83.63170945779077670, -296.0521521680024080, -417.1172536214571096 ) ) ;
#45424=CARTESIAN_POINT ( 'NONE',  ( 113.5000000000000568, -218.8335761803644743, -447.4016117689005796 ) ) ;
#45702=VERTEX_POINT ( 'NONE', #52088 ) ;
#45791=CARTESIAN_POINT ( 'NONE',  ( 113.5000000000000568, -190.7866584945343504, -447.4016117689005796 ) ) ;
#45814=ADVANCED_FACE ( 'NONE', ( #15643 ), #1432, .F. ) ;
#46038=LINE ( 'NONE', #10053, #2323 ) ;
#46184=EDGE_CURVE ( 'NONE', #66186, #26725, #81420, .T. ) ;
#46260=LINE ( 'NONE', #89336, #39844 ) ;
#46279=DIRECTION ( 'NONE',  ( 0.000000000000000000, 0.000000000000000000, 1.000000000000000000 ) ) ;
#46500=ORIENTED_EDGE ( 'NONE', *, *, #61310, .F. ) ;
#46641=DIRECTION ( 'NONE',  ( 0.000000000000000000, -1.000000000000000000, 0.000000000000000000 ) ) ;
#46848=ORIENTED_EDGE ( 'NONE', *, *, #65933, .T. ) ;
#46978=DIRECTION ( 'NONE',  ( -0.000000000000000000, 1.000000000000000000, -0.000000000000000000 ) ) ;
#47034=EDGE_CURVE ( 'NONE', #77282, #16610, #90665, .T. ) ;
#47147=AXIS2_PLACEMENT_3D ( 'NONE', #53320, #61842, #40952 ) ;
#47174=DIRECTION ( 'NONE',  ( 0.000000000000000000, 0.000000000000000000, 1.000000000000000000 ) ) ;
#47269=VECTOR ( 'NONE', #47921, 1000.000000000000000 ) ;
#47355=DIRECTION ( 'NONE',  ( -0.000000000000000000, 1.000000000000000000, -0.000000000000000000 ) ) ;
#47581=VECTOR ( 'NONE', #64745, 1000.000000000000114 ) ;
#47636=EDGE_CURVE ( 'NONE', #74793, #66186, #22928, .T. ) ;
#47639=ORIENTED_EDGE ( 'NONE', *, *, #89695, .T. ) ;
#47780=VECTOR ( 'NONE', #90276, 1000.000000000000000 ) ;
#47921=DIRECTION ( 'NONE',  ( 0.000000000000000000, 0.000000000000000000, -1.000000000000000000 ) ) ;
#47975=VERTEX_POINT ( 'NONE', #74515 ) ;
#48006=ORIENTED_EDGE ( 'NONE', *, *, #33276, .F. ) ;
#48217=EDGE_CURVE ( 'NONE', #66186, #62642, #48904, .T. ) ;
#48421=EDGE_LOOP ( 'NONE', ( #57904, #76580, #91691, #85614 ) ) ;
#48424=CARTESIAN_POINT ( 'NONE',  ( 113.5000000000000568, -298.0521521680024080, -397.9547385950631337 ) ) ;
#48447=LINE ( 'NONE', #68376, #8035 ) ;
#48552=DIRECTION ( 'NONE',  ( 1.000000000000000000, 0.000000000000000000, -0.000000000000000000 ) ) ;
#48748=ORIENTED_EDGE ( 'NONE', *, *, #4833, .T. ) ;
#48834=SHAPE_REPRESENTATION_RELATIONSHIP ( 'NONE' , 'NONE' ,  #61554, #75750 ) ;
#48875=CARTESIAN_POINT ( 'NONE',  ( 85.55100297371609486, -298.0521521680024080, -525.1711561948568487 ) ) ;
#48904=LINE ( 'NONE', #48424, #7427 ) ;
#49040=DIRECTION ( 'NONE',  ( -0.000000000000000000, 1.000000000000000000, 0.000000000000000000 ) ) ;
#49234=DIRECTION ( 'NONE',  ( 0.000000000000000000, 0.9681751575201845705, -0.2502735790305593011 ) ) ;
#49342=VERTEX_POINT ( 'NONE', #57435 ) ;
#49476=CARTESIAN_POINT ( 'NONE',  ( -83.63170945779077670, -298.0521521680024080, -417.1172536214571096 ) ) ;
#49483=FACE_OUTER_BOUND ( 'NONE', #69338, .T. ) ;
#49566=CARTESIAN_POINT ( 'NONE',  ( -113.5000000000000568, -296.0521521680024080, -537.7509286889328450 ) ) ;
#49622=FACE_OUTER_BOUND ( 'NONE', #76816, .T. ) ;
#49869=DIRECTION ( 'NONE',  ( 0.000000000000000000, 0.000000000000000000, 1.000000000000000000 ) ) ;
#50051=FACE_BOUND ( 'NONE', #85089, .T. ) ;
#50117=( NAMED_UNIT ( * ) SI_UNIT ( $, .STERADIAN. ) SOLID_ANGLE_UNIT ( ) );
#50140=AXIS2_PLACEMENT_3D ( 'NONE', #40834, #91514, #3014 ) ;
#50161=EDGE_CURVE ( 'NONE', #77282, #32191, #55899, .T. ) ;
#50708=PRODUCT_DEFINITION_FORMATION_WITH_SPECIFIED_SOURCE ( 'ANY', '', #1958, .NOT_KNOWN. ) ;
#50987=DIRECTION ( 'NONE',  ( -0.000000000000000000, 1.000000000000000000, 0.000000000000000000 ) ) ;
#51112=DIRECTION ( 'NONE',  ( 0.000000000000000000, 0.000000000000000000, 1.000000000000000000 ) ) ;
#51278=ORIENTED_EDGE ( 'NONE', *, *, #13868, .T. ) ;
#51686=CARTESIAN_POINT ( 'NONE',  ( -113.5000000000000568, -218.8335761803644743, -490.8867980474134356 ) ) ;
#52088=CARTESIAN_POINT ( 'NONE',  ( 113.5000000000000568, -212.3147208684173108, -422.1836331355066818 ) ) ;
#52109=ORIENTED_EDGE ( 'NONE', *, *, #88840, .F. ) ;
#52151=CARTESIAN_POINT ( 'NONE',  ( 85.55100297371598117, -296.0521521680024080, -413.1172536214571096 ) ) ;
#52541=ORIENTED_EDGE ( 'NONE', *, *, #83711, .F. ) ;
#52591=CARTESIAN_POINT ( 'NONE',  ( 113.5000000000000568, -190.7866584945343504, -447.4016117689005796 ) ) ;
#52941=CARTESIAN_POINT ( 'NONE',  ( 113.5000000000000568, -218.8335761803644743, -490.8867980474134356 ) ) ;
#53320=CARTESIAN_POINT ( 'NONE',  ( -83.63170945779074827, -298.0521521680024080, -521.1711561948568487 ) ) ;
#53579=ORIENTED_EDGE ( 'NONE', *, *, #55666, .T. ) ;
#53688=DIRECTION ( 'NONE',  ( -0.000000000000000000, -0.9681751575201845705, 0.2502735790305594676 ) ) ;
#53772=FACE_OUTER_BOUND ( 'NONE', #39966, .T. ) ;
#53801=DIRECTION ( 'NONE',  ( -0.000000000000000000, 1.000000000000000000, 0.000000000000000000 ) ) ;
#53945=EDGE_LOOP ( 'NONE', ( #41645, #91946 ) ) ;
#54562=CARTESIAN_POINT ( 'NONE',  ( 113.5000000000000568, -296.0521521680024080, -400.5374811273811702 ) ) ;
#54768=LINE ( 'NONE', #45791, #88600 ) ;
#54788=CARTESIAN_POINT ( 'NONE',  ( 85.55100297371598117, -296.0521521680024080, -417.1172536214571096 ) ) ;
#54874=EDGE_CURVE ( 'NONE', #28339, #32344, #37881, .T. ) ;
#55159=ORIENTED_EDGE ( 'NONE', *, *, #4833, .F. ) ;
#55318=AXIS2_PLACEMENT_3D ( 'NONE', #29188, #67035, #36285 ) ;
#55666=EDGE_CURVE ( 'NONE', #36954, #83022, #57014, .T. ) ;
#55671=DIRECTION ( 'NONE',  ( -1.000000000000000000, -0.000000000000000000, -0.000000000000000000 ) ) ;
#55768=AXIS2_PLACEMENT_3D ( 'NONE', #44513, #1900, #74325 ) ;
#55885=DIRECTION ( 'NONE',  ( -0.000000000000000000, 1.000000000000000000, -0.000000000000000000 ) ) ;
#55899=CIRCLE ( 'NONE', #78549, 4.000000000000003553 ) ;
#56009=CARTESIAN_POINT ( 'NONE',  ( 85.55100297371609486, -373.0521521680024648, -521.1711561948568487 ) ) ;
#56311=( NAMED_UNIT ( * ) PLANE_ANGLE_UNIT ( ) SI_UNIT ( $, .RADIAN. ) );
#56322=ADVANCED_FACE ( 'NONE', ( #72144 ), #36137, .F. ) ;
#56466=LINE ( 'NONE', #11004, #6492 ) ;
#56468=AXIS2_PLACEMENT_3D ( 'NONE', #54788, #10768, #74723 ) ;
#56602=VECTOR ( 'NONE', #74283, 1000.000000000000000 ) ;
#56694=AXIS2_PLACEMENT_3D ( 'NONE', #45424, #73866, #75266 ) ;
#56884=ORIENTED_EDGE ( 'NONE', *, *, #13868, .F. ) ;
#56922=VERTEX_POINT ( 'NONE', #35912 ) ;
#57014=LINE ( 'NONE', #85850, #81760 ) ;
#57089=CARTESIAN_POINT ( 'NONE',  ( 113.5000000000000568, -190.7866584945343504, -447.4016117689005796 ) ) ;
#57136=ADVANCED_FACE ( 'NONE', ( #78078, #34975, #14616, #42530, #78540 ), #63889, .T. ) ;
#57164=CARTESIAN_POINT ( 'NONE',  ( -113.5000000000000568, -190.7866584945343220, -490.8867980474134356 ) ) ;
#57340=EDGE_CURVE ( 'NONE', #37982, #91222, #1316, .T. ) ;
#57412=CIRCLE ( 'NONE', #92178, 4.000000000000003553 ) ;
#57427=LINE ( 'NONE', #78723, #12668 ) ;
#57435=CARTESIAN_POINT ( 'NONE',  ( -83.63170945779074827, -296.0521521680024080, -517.1711561948568487 ) ) ;
#57449=ORIENTED_EDGE ( 'NONE', *, *, #13625, .F. ) ;
#57556=CARTESIAN_POINT ( 'NONE',  ( 85.55100297371609486, -298.0521521680024080, -517.1711561948568487 ) ) ;
#57559=ADVANCED_FACE ( 'NONE', ( #89804 ), #24482, .F. ) ;
#57627=ORIENTED_EDGE ( 'NONE', *, *, #34351, .T. ) ;
#57904=ORIENTED_EDGE ( 'NONE', *, *, #92091, .T. ) ;
#57947=ORIENTED_EDGE ( 'NONE', *, *, #36806, .T. ) ;
#58278=CARTESIAN_POINT ( 'NONE',  ( 85.55100297371598117, -298.0521521680024080, -417.1172536214571096 ) ) ;
#58384=ADVANCED_FACE ( 'NONE', ( #11985 ), #90555, .F. ) ;
#58628=CARTESIAN_POINT ( 'NONE',  ( 113.5000000000000568, -296.0521521680024080, -537.7509286889328450 ) ) ;
#58675=DIRECTION ( 'NONE',  ( 1.000000000000000000, 0.000000000000000000, 0.000000000000000000 ) ) ;
#58850=DIRECTION ( 'NONE',  ( -0.000000000000000000, 1.000000000000000000, -0.000000000000000000 ) ) ;
#59201=VERTEX_POINT ( 'NONE', #59279 ) ;
#59215=CIRCLE ( 'NONE', #18379, 26.04691768583017364 ) ;
#59245=ORIENTED_EDGE ( 'NONE', *, *, #68227, .T. ) ;
#59279=CARTESIAN_POINT ( 'NONE',  ( -83.63170945779077670, -298.0521521680024080, -413.1172536214571096 ) ) ;
#59329=VERTEX_POINT ( 'NONE', #24202 ) ;
#59350=VECTOR ( 'NONE', #30154, 1000.000000000000000 ) ;
#59412=AXIS2_PLACEMENT_3D ( 'NONE', #67857, #46978, #9134 ) ;
#59451=VERTEX_POINT ( 'NONE', #74884 ) ;
#59580=ORIENTED_EDGE ( 'NONE', *, *, #16109, .F. ) ;
#60019=DIRECTION ( 'NONE',  ( -0.000000000000000000, -0.9681751575201845705, 0.2502735790305593011 ) ) ;
#60045=ORIENTED_EDGE ( 'NONE', *, *, #35632, .T. ) ;
#60146=DIRECTION ( 'NONE',  ( -1.000000000000000000, -0.000000000000000000, -0.000000000000000000 ) ) ;
#60203=EDGE_CURVE ( 'NONE', #92631, #59201, #71454, .T. ) ;
#60401=EDGE_LOOP ( 'NONE', ( #14078, #48006, #88344, #74016 ) ) ;
#60445=DIRECTION ( 'NONE',  ( 0.000000000000000000, 1.000000000000000000, 0.000000000000000000 ) ) ;
#60519=CARTESIAN_POINT ( 'NONE',  ( -113.5000000000000568, -218.8335761803644743, -447.4016117689005796 ) ) ;
#60619=ORIENTED_EDGE ( 'NONE', *, *, #47636, .T. ) ;
#60847=EDGE_LOOP ( 'NONE', ( #61207, #52541 ) ) ;
#60916=CARTESIAN_POINT ( 'NONE',  ( -83.63170945779074827, -298.0521521680024080, -521.1711561948568487 ) ) ;
#61207=ORIENTED_EDGE ( 'NONE', *, *, #22793, .F. ) ;
#61310=EDGE_CURVE ( 'NONE', #12065, #83022, #68486, .T. ) ;
#61312=DIRECTION ( 'NONE',  ( 0.000000000000000000, 0.000000000000000000, -1.000000000000000000 ) ) ;
#61365=DIRECTION ( 'NONE',  ( 0.000000000000000000, -0.000000000000000000, -1.000000000000000000 ) ) ;
#61458=EDGE_LOOP ( 'NONE', ( #417, #33131, #26753, #29531, #77486, #62844 ) ) ;
#61554=SHAPE_REPRESENTATION ( 'Metal Foot Protection Guard', ( #18940 ), #91438 ) ;
#61842=DIRECTION ( 'NONE',  ( -0.000000000000000000, 1.000000000000000000, 0.000000000000000000 ) ) ;
#61914=LINE ( 'NONE', #83669, #77519 ) ;
#61996=EDGE_LOOP ( 'NONE', ( #18420, #43838 ) ) ;
#62010=ORIENTED_EDGE ( 'NONE', *, *, #60203, .F. ) ;
#62083=EDGE_CURVE ( 'NONE', #59329, #36642, #61914, .T. ) ;
#62128=DIRECTION ( 'NONE',  ( -0.000000000000000000, -0.9681751575201845705, 0.2502735790305593011 ) ) ;
#62147=EDGE_LOOP ( 'NONE', ( #60619, #69652, #43156, #46848, #28860, #69963 ) ) ;
#62368=VERTEX_POINT ( 'NONE', #57164 ) ;
#62468=VERTEX_POINT ( 'NONE', #33970 ) ;
#62642=VERTEX_POINT ( 'NONE', #93574 ) ;
#62844=ORIENTED_EDGE ( 'NONE', *, *, #83939, .F. ) ;
#62854=CARTESIAN_POINT ( 'NONE',  ( -113.5000000000000568, -192.7866584945343504, -490.8867980474134356 ) ) ;
#63002=ORIENTED_EDGE ( 'NONE', *, *, #74417, .F. ) ;
#63024=ADVANCED_FACE ( 'NONE', ( #81122 ), #17200, .F. ) ;
#63088=( NAMED_UNIT ( * ) SI_UNIT ( $, .STERADIAN. ) SOLID_ANGLE_UNIT ( ) );
#63142=FACE_OUTER_BOUND ( 'NONE', #89467, .T. ) ;
#63148=FACE_OUTER_BOUND ( 'NONE', #88219, .T. ) ;
#63245=DIRECTION ( 'NONE',  ( -0.000000000000000000, 1.000000000000000000, 0.000000000000000000 ) ) ;
#63400=DIRECTION ( 'NONE',  ( 0.000000000000000000, 0.000000000000000000, 1.000000000000000000 ) ) ;
#63556=EDGE_CURVE ( 'NONE', #56922, #37982, #19066, .T. ) ;
#63681=EDGE_CURVE ( 'NONE', #93231, #36642, #56466, .T. ) ;
#63889=PLANE ( 'NONE',  #36491 ) ;
#63892=CARTESIAN_POINT ( 'NONE',  ( 85.55100297371609486, -373.0521521680024648, -525.1711561948568487 ) ) ;
#64302=ORIENTED_EDGE ( 'NONE', *, *, #27474, .F. ) ;
#64306=ADVANCED_FACE ( 'NONE', ( #31299 ), #81462, .F. ) ;
#64374=CARTESIAN_POINT ( 'NONE',  ( 113.5000000000000568, -296.0521521680024080, -400.5374811273811702 ) ) ;
#64564=DIRECTION ( 'NONE',  ( -0.000000000000000000, 1.000000000000000000, -0.000000000000000000 ) ) ;
#64644=EDGE_LOOP ( 'NONE', ( #9540, #1878, #69540, #85542, #41963, #48748 ) ) ;
#64676=DIRECTION ( 'NONE',  ( 0.000000000000000000, -0.000000000000000000, -1.000000000000000000 ) ) ;
#64745=DIRECTION ( 'NONE',  ( 0.000000000000000000, 0.9681751575201842375, 0.2502735790305606889 ) ) ;
#64793=CIRCLE ( 'NONE', #93474, 28.04691768583012035 ) ;
#64844=LINE ( 'NONE', #30209, #38600 ) ;
#64959=ORIENTED_EDGE ( 'NONE', *, *, #50161, .T. ) ;
#65051=CARTESIAN_POINT ( 'NONE',  ( -83.63170945779077670, -373.0521521680024648, -413.1172536214571096 ) ) ;
#65128=DIRECTION ( 'NONE',  ( 0.000000000000000000, 0.000000000000000000, 1.000000000000000000 ) ) ;
#65205=FACE_BOUND ( 'NONE', #64644, .T. ) ;
#65231=CARTESIAN_POINT ( 'NONE',  ( -113.5000000000000568, -190.7866584945343504, -447.4016117689005796 ) ) ;
#65404=ADVANCED_FACE ( 'NONE', ( #42580 ), #79529, .T. ) ;
#65512=DIRECTION ( 'NONE',  ( 0.000000000000000000, 0.9681751575201845705, 0.2502735790305594676 ) ) ;
#65769=LINE ( 'NONE', #9340, #38727 ) ;
#65933=EDGE_CURVE ( 'NONE', #12065, #47975, #44313, .T. ) ;
#66156=LINE ( 'NONE', #32008, #59350 ) ;
#66186=VERTEX_POINT ( 'NONE', #77063 ) ;
#66271=DIRECTION ( 'NONE',  ( -0.000000000000000000, 1.000000000000000000, -0.000000000000000000 ) ) ;
#66472=ORIENTED_EDGE ( 'NONE', *, *, #17028, .T. ) ;
#66807=DIRECTION ( 'NONE',  ( 0.000000000000000000, -0.2502735790305594676, -0.9681751575201846816 ) ) ;
#66844=DIRECTION ( 'NONE',  ( 0.000000000000000000, 0.000000000000000000, 1.000000000000000000 ) ) ;
#66969=AXIS2_PLACEMENT_3D ( 'NONE', #92547, #27715, #71753 ) ;
#67035=DIRECTION ( 'NONE',  ( -1.000000000000000000, -0.000000000000000000, 0.000000000000000000 ) ) ;
#67111=ORIENTED_EDGE ( 'NONE', *, *, #73397, .T. ) ;
#67191=CARTESIAN_POINT ( 'NONE',  ( 85.55100297371609486, -296.0521521680024080, -521.1711561948568487 ) ) ;
#67249=CARTESIAN_POINT ( 'NONE',  ( 113.5000000000000568, -298.0521521680024080, -397.9547385950631337 ) ) ;
#67787=ADVANCED_FACE ( 'NONE', ( #53772 ), #69374, .T. ) ;
#67857=CARTESIAN_POINT ( 'NONE',  ( 85.55100297371598117, -373.0521521680024648, -417.1172536214571096 ) ) ;
#68059=DIRECTION ( 'NONE',  ( -0.000000000000000000, -0.000000000000000000, 1.000000000000000000 ) ) ;
#68227=EDGE_CURVE ( 'NONE', #59201, #92631, #20278, .T. ) ;
#68307=CARTESIAN_POINT ( 'NONE',  ( -113.5000000000000568, -218.8335761803644743, -490.8867980474134356 ) ) ;
#68326=EDGE_LOOP ( 'NONE', ( #85632, #5173, #1936, #82606 ) ) ;
#68376=CARTESIAN_POINT ( 'NONE',  ( -113.5000000000000568, -296.0521521680024080, -400.5374811273811702 ) ) ;
#68486=LINE ( 'NONE', #39107, #29126 ) ;
#68705=DIRECTION ( 'NONE',  ( 0.000000000000000000, 0.000000000000000000, -1.000000000000000000 ) ) ;
#69096=EDGE_LOOP ( 'NONE', ( #85442, #40514, #19877, #84931 ) ) ;
#69338=EDGE_LOOP ( 'NONE', ( #16152, #11572, #85318, #60045 ) ) ;
#69374=PLANE ( 'NONE',  #24795 ) ;
#69395=CARTESIAN_POINT ( 'NONE',  ( 113.5000000000000568, -212.3147208684173108, -422.1836331355066818 ) ) ;
#69540=ORIENTED_EDGE ( 'NONE', *, *, #93458, .T. ) ;
#69640=CARTESIAN_POINT ( 'NONE',  ( -113.5000000000000568, -296.0521521680024080, -400.5374811273811702 ) ) ;
#69652=ORIENTED_EDGE ( 'NONE', *, *, #48217, .T. ) ;
#69750=DIRECTION ( 'NONE',  ( -0.000000000000000000, 1.000000000000000000, -0.000000000000000000 ) ) ;
#69956=VECTOR ( 'NONE', #83118, 1000.000000000000000 ) ;
#69963=ORIENTED_EDGE ( 'NONE', *, *, #44156, .T. ) ;
#70096=DIRECTION ( 'NONE',  ( 0.000000000000000000, 0.000000000000000000, 1.000000000000000000 ) ) ;
#70105=PRODUCT_DEFINITION_SHAPE ( 'NONE', 'NONE',  #19232 ) ;
#70329=UNCERTAINTY_MEASURE_WITH_UNIT (LENGTH_MEASURE( 1.000000000000000082E-05 ), #7172, 'distance_accuracy_value', 'NONE');
#70339=CIRCLE ( 'NONE', #83953, 28.04691768583012035 ) ;
#70405=( GEOMETRIC_REPRESENTATION_CONTEXT ( 3 ) GLOBAL_UNCERTAINTY_ASSIGNED_CONTEXT ( ( #4574 ) ) GLOBAL_UNIT_ASSIGNED_CONTEXT ( ( #34987, #56311, #50117 ) ) REPRESENTATION_CONTEXT ( 'NONE', 'WORKASPACE' ) );
#70563=ORIENTED_EDGE ( 'NONE', *, *, #40622, .T. ) ;
#71098=ORIENTED_EDGE ( 'NONE', *, *, #3235, .F. ) ;
#71251=ORIENTED_EDGE ( 'NONE', *, *, #27503, .F. ) ;
#71274=CARTESIAN_POINT ( 'NONE',  ( 113.5000000000000568, -296.0521521680024080, -537.7509286889328450 ) ) ;
#71285=DIRECTION ( 'NONE',  ( 0.000000000000000000, -1.000000000000000000, 0.000000000000000000 ) ) ;
#71340=DIRECTION ( 'NONE',  ( -1.000000000000000000, -0.000000000000000000, -0.000000000000000000 ) ) ;
#71344=EDGE_LOOP ( 'NONE', ( #55159, #37901, #80900, #81056 ) ) ;
#71390=CARTESIAN_POINT ( 'NONE',  ( 113.5000000000000568, -298.0521521680024080, -397.9547385950631337 ) ) ;
#71431=CARTESIAN_POINT ( 'NONE',  ( -113.5000000000000568, -211.8141737103562434, -518.0411269958476623 ) ) ;
#71454=CIRCLE ( 'NONE', #91058, 4.000000000000003553 ) ;
#71495=DIRECTION ( 'NONE',  ( 0.000000000000000000, -0.2502735790305593566, -0.9681751575201846816 ) ) ;
#71705=ADVANCED_FACE ( 'NONE', ( #78489, #6987, #50051, #93145, #14096 ), #6052, .F. ) ;
#71753=DIRECTION ( 'NONE',  ( 0.000000000000000000, 0.000000000000000000, 1.000000000000000000 ) ) ;
#71921=DIRECTION ( 'NONE',  ( 0.000000000000000000, -0.000000000000000000, 1.000000000000000000 ) ) ;
#72103=DIRECTION ( 'NONE',  ( -1.000000000000000000, -0.000000000000000000, -0.000000000000000000 ) ) ;
#72116=CARTESIAN_POINT ( 'NONE',  ( 113.5000000000000568, -212.3147208684173677, -516.1047766808072765 ) ) ;
#72144=FACE_OUTER_BOUND ( 'NONE', #71344, .T. ) ;
#72178=ORIENTED_EDGE ( 'NONE', *, *, #32846, .F. ) ;
#72303=EDGE_CURVE ( 'NONE', #37982, #28339, #9758, .T. ) ;
#72405=VECTOR ( 'NONE', #72669, 1000.000000000000000 ) ;
#72669=DIRECTION ( 'NONE',  ( -0.000000000000000000, 1.000000000000000000, -0.000000000000000000 ) ) ;
#73286=CIRCLE ( 'NONE', #11220, 26.04691768583011680 ) ;
#73301=AXIS2_PLACEMENT_3D ( 'NONE', #90372, #77131, #17968 ) ;
#73397=EDGE_CURVE ( 'NONE', #49342, #81684, #57412, .T. ) ;
#73466=CARTESIAN_POINT ( 'NONE',  ( 113.5000000000000568, -192.7866584945343504, -490.8867980474134356 ) ) ;
#73595=DIRECTION ( 'NONE',  ( 0.000000000000000000, 1.000000000000000000, -0.000000000000000000 ) ) ;
#73755=DIRECTION ( 'NONE',  ( -1.000000000000000000, -0.000000000000000000, -0.000000000000000000 ) ) ;
#73866=DIRECTION ( 'NONE',  ( -1.000000000000000000, -0.000000000000000000, 0.000000000000000000 ) ) ;
#74016=ORIENTED_EDGE ( 'NONE', *, *, #25097, .T. ) ;
#74067=AXIS2_PLACEMENT_3D ( 'NONE', #35165, #64564, #77325 ) ;
#74256=ORIENTED_EDGE ( 'NONE', *, *, #36806, .F. ) ;
#74283=DIRECTION ( 'NONE',  ( -0.000000000000000000, 1.000000000000000000, -0.000000000000000000 ) ) ;
#74325=DIRECTION ( 'NONE',  ( 0.000000000000000000, 0.000000000000000000, 1.000000000000000000 ) ) ;
#74329=VECTOR ( 'NONE', #73755, 1000.000000000000000 ) ;
#74417=EDGE_CURVE ( 'NONE', #11793, #81684, #33765, .T. ) ;
#74465=AXIS2_PLACEMENT_3D ( 'NONE', #38642, #60445, #75109 ) ;
#74515=CARTESIAN_POINT ( 'NONE',  ( 113.5000000000000568, -190.7866584945343220, -490.8867980474134356 ) ) ;
#74600=AXIS2_PLACEMENT_3D ( 'NONE', #71390, #50987, #79427 ) ;
#74723=DIRECTION ( 'NONE',  ( 0.000000000000000000, 0.000000000000000000, -1.000000000000000000 ) ) ;
#74793=VERTEX_POINT ( 'NONE', #75452 ) ;
#74863=DIRECTION ( 'NONE',  ( -1.000000000000000000, -0.000000000000000000, -0.000000000000000000 ) ) ;
#74884=CARTESIAN_POINT ( 'NONE',  ( -113.5000000000000568, -212.3147208684173108, -422.1836331355066818 ) ) ;
#74931=ADVANCED_FACE ( 'NONE', ( #63148 ), #77802, .F. ) ;
#75109=DIRECTION ( 'NONE',  ( 0.000000000000000000, 0.000000000000000000, 1.000000000000000000 ) ) ;
#75266=DIRECTION ( 'NONE',  ( 0.000000000000000000, 0.000000000000000000, 1.000000000000000000 ) ) ;
#75452=CARTESIAN_POINT ( 'NONE',  ( 113.5000000000000568, -211.8141737103562434, -420.2472828204663529 ) ) ;
#75750=ADVANCED_BREP_SHAPE_REPRESENTATION ( '', ( #91220, #18940 ), #91438 ) ;
#75779=LINE ( 'NONE', #24656, #9664 ) ;
#76110=EDGE_LOOP ( 'NONE', ( #57947, #24218, #5158, #28110 ) ) ;
#76222=SHAPE_DEFINITION_REPRESENTATION ( #70105, #61554 ) ;
#76580=ORIENTED_EDGE ( 'NONE', *, *, #46184, .F. ) ;
#76734=LINE ( 'NONE', #18490, #23184 ) ;
#76758=ORIENTED_EDGE ( 'NONE', *, *, #47034, .F. ) ;
#76816=EDGE_LOOP ( 'NONE', ( #18585, #38918, #38490, #56884 ) ) ;
#76975=EDGE_CURVE ( 'NONE', #32191, #77282, #28804, .T. ) ;
#77063=CARTESIAN_POINT ( 'NONE',  ( 113.5000000000000568, -298.0521521680024080, -397.9547385950631337 ) ) ;
#77131=DIRECTION ( 'NONE',  ( 0.000000000000000000, -0.2502735790305594676, 0.9681751575201846816 ) ) ;
#77187=CYLINDRICAL_SURFACE ( 'NONE', #26374, 4.000000000000003553 ) ;
#77199=LINE ( 'NONE', #19434, #42989 ) ;
#77265=( NAMED_UNIT ( * ) PLANE_ANGLE_UNIT ( ) SI_UNIT ( $, .RADIAN. ) );
#77282=VERTEX_POINT ( 'NONE', #57556 ) ;
#77325=DIRECTION ( 'NONE',  ( 0.000000000000000000, 0.000000000000000000, 1.000000000000000000 ) ) ;
#77456=DIRECTION ( 'NONE',  ( -0.000000000000000000, 1.000000000000000000, 0.000000000000000000 ) ) ;
#77460=CIRCLE ( 'NONE', #83452, 28.04691768583012035 ) ;
#77486=ORIENTED_EDGE ( 'NONE', *, *, #63556, .F. ) ;
#77519=VECTOR ( 'NONE', #10301, 1000.000000000000000 ) ;
#77613=CIRCLE ( 'NONE', #8052, 4.000000000000003553 ) ;
#77662=DIRECTION ( 'NONE',  ( 0.000000000000000000, 0.000000000000000000, 1.000000000000000000 ) ) ;
#77802=CYLINDRICAL_SURFACE ( 'NONE', #74067, 4.000000000000003553 ) ;
#77918=CARTESIAN_POINT ( 'NONE',  ( -83.63170945779074827, -296.0521521680024080, -521.1711561948568487 ) ) ;
#78000=EDGE_LOOP ( 'NONE', ( #59245, #85997 ) ) ;
#78078=FACE_BOUND ( 'NONE', #53945, .T. ) ;
#78364=APPLICATION_CONTEXT ( 'automotive_design' ) ;
#78384=DIRECTION ( 'NONE',  ( -1.000000000000000000, -0.000000000000000000, -0.000000000000000000 ) ) ;
#78396=CARTESIAN_POINT ( 'NONE',  ( 85.55100297371609486, -298.0521521680024080, -521.1711561948568487 ) ) ;
#78489=FACE_BOUND ( 'NONE', #34433, .T. ) ;
#78540=FACE_OUTER_BOUND ( 'NONE', #68326, .T. ) ;
#78549=AXIS2_PLACEMENT_3D ( 'NONE', #84078, #77456, #12119 ) ;
#78723=CARTESIAN_POINT ( 'NONE',  ( 113.5000000000000568, -212.3147208684173677, -516.1047766808072765 ) ) ;
#78843=LINE ( 'NONE', #35763, #15682 ) ;
#78948=CIRCLE ( 'NONE', #47147, 4.000000000000003553 ) ;
#79019=VECTOR ( 'NONE', #55671, 1000.000000000000000 ) ;
#79083=AXIS2_PLACEMENT_3D ( 'NONE', #71274, #6401, #35273 ) ;
#79325=VECTOR ( 'NONE', #58850, 1000.000000000000000 ) ;
#79427=DIRECTION ( 'NONE',  ( 0.000000000000000000, -0.000000000000000000, 1.000000000000000000 ) ) ;
#79529=PLANE ( 'NONE',  #92713 ) ;
#79554=LINE ( 'NONE', #21313, #11217 ) ;
#79851=CARTESIAN_POINT ( 'NONE',  ( 113.5000000000000568, -298.0521521680024080, -540.3336712212508246 ) ) ;
#80428=DIRECTION ( 'NONE',  ( 0.000000000000000000, 0.000000000000000000, -1.000000000000000000 ) ) ;
#80681=CARTESIAN_POINT ( 'NONE',  ( 85.55100297371598117, -296.0521521680024080, -417.1172536214571096 ) ) ;
#80738=EDGE_CURVE ( 'NONE', #2276, #24966, #9526, .T. ) ;
#80865=CARTESIAN_POINT ( 'NONE',  ( 113.5000000000000568, -192.7866584945343504, -447.4016117689005796 ) ) ;
#80900=ORIENTED_EDGE ( 'NONE', *, *, #54874, .T. ) ;
#80903=AXIS2_PLACEMENT_3D ( 'NONE', #91285, #41569, #63400 ) ;
#81056=ORIENTED_EDGE ( 'NONE', *, *, #27503, .T. ) ;
#81122=FACE_OUTER_BOUND ( 'NONE', #18451, .T. ) ;
#81159=CARTESIAN_POINT ( 'NONE',  ( 113.5000000000000568, -211.8141737103562434, -518.0411269958476623 ) ) ;
#81420=LINE ( 'NONE', #67249, #8832 ) ;
#81462=PLANE ( 'NONE',  #2011 ) ;
#81507=ORIENTED_EDGE ( 'NONE', *, *, #61310, .T. ) ;
#81543=ORIENTED_EDGE ( 'NONE', *, *, #80738, .F. ) ;
#81684=VERTEX_POINT ( 'NONE', #23194 ) ;
#81760=VECTOR ( 'NONE', #65512, 1000.000000000000227 ) ;
#82454=ORIENTED_EDGE ( 'NONE', *, *, #76975, .T. ) ;
#82606=ORIENTED_EDGE ( 'NONE', *, *, #57340, .T. ) ;
#82789=DIRECTION ( 'NONE',  ( -0.000000000000000000, 1.000000000000000000, 0.000000000000000000 ) ) ;
#82940=ORIENTED_EDGE ( 'NONE', *, *, #12809, .T. ) ;
#83022=VERTEX_POINT ( 'NONE', #71431 ) ;
#83095=CARTESIAN_POINT ( 'NONE',  ( 113.5000000000000568, -192.7866584945343504, -447.4016117689005796 ) ) ;
#83118=DIRECTION ( 'NONE',  ( -1.000000000000000000, -0.000000000000000000, -0.000000000000000000 ) ) ;
#83158=APPLICATION_CONTEXT ( 'automotive_design' ) ;
#83179=DIRECTION ( 'NONE',  ( -0.000000000000000000, -0.9681751575201845705, 0.2502735790305594676 ) ) ;
#83344=CARTESIAN_POINT ( 'NONE',  ( -113.5000000000000568, -298.0521521680024080, -397.9547385950631337 ) ) ;
#83452=AXIS2_PLACEMENT_3D ( 'NONE', #51686, #28547, #26790 ) ;
#83669=CARTESIAN_POINT ( 'NONE',  ( 113.5000000000000568, -192.7866584945343504, -447.4016117689005796 ) ) ;
#83711=EDGE_CURVE ( 'NONE', #9616, #29874, #11159, .T. ) ;
#83939=EDGE_CURVE ( 'NONE', #45702, #56922, #2249, .T. ) ;
#83953=AXIS2_PLACEMENT_3D ( 'NONE', #60519, #32571, #46279 ) ;
#84078=CARTESIAN_POINT ( 'NONE',  ( 85.55100297371609486, -298.0521521680024080, -521.1711561948568487 ) ) ;
#84286=CARTESIAN_POINT ( 'NONE',  ( -113.5000000000000568, -192.7866584945343504, -447.4016117689005796 ) ) ;
#84428=ORIENTED_EDGE ( 'NONE', *, *, #11459, .T. ) ;
#84503=DIRECTION ( 'NONE',  ( 0.000000000000000000, 0.000000000000000000, 1.000000000000000000 ) ) ;
#84536=CARTESIAN_POINT ( 'NONE',  ( 113.5000000000000568, -218.8335761803644743, -447.4016117689005796 ) ) ;
#84617=EDGE_CURVE ( 'NONE', #59201, #29874, #29034, .T. ) ;
#84931=ORIENTED_EDGE ( 'NONE', *, *, #41482, .T. ) ;
#85054=CYLINDRICAL_SURFACE ( 'NONE', #27811, 28.04691768583012035 ) ;
#85089=EDGE_LOOP ( 'NONE', ( #70563, #66472 ) ) ;
#85241=CARTESIAN_POINT ( 'NONE',  ( -113.5000000000000568, -298.0521521680024080, -540.3336712212508246 ) ) ;
#85318=ORIENTED_EDGE ( 'NONE', *, *, #72303, .T. ) ;
#85442=ORIENTED_EDGE ( 'NONE', *, *, #87369, .F. ) ;
#85542=ORIENTED_EDGE ( 'NONE', *, *, #9353, .T. ) ;
#85614=ORIENTED_EDGE ( 'NONE', *, *, #37532, .T. ) ;
#85632=ORIENTED_EDGE ( 'NONE', *, *, #9353, .F. ) ;
#85658=EDGE_LOOP ( 'NONE', ( #62010, #19258, #10078, #28573 ) ) ;
#85850=CARTESIAN_POINT ( 'NONE',  ( -113.5000000000000568, -298.0521521680024080, -540.3336712212508246 ) ) ;
#85997=ORIENTED_EDGE ( 'NONE', *, *, #60203, .T. ) ;
#86201=ADVANCED_FACE ( 'NONE', ( #32177, #24130 ), #17038, .F. ) ;
#86290=VERTEX_POINT ( 'NONE', #39248 ) ;
#86365=AXIS2_PLACEMENT_3D ( 'NONE', #37511, #1539, #49869 ) ;
#86465=LINE ( 'NONE', #79851, #15544 ) ;
#86552=CIRCLE ( 'NONE', #38221, 4.000000000000003553 ) ;
#86631=AXIS2_PLACEMENT_3D ( 'NONE', #15729, #30870, #66844 ) ;
#86799=ORIENTED_EDGE ( 'NONE', *, *, #89695, .F. ) ;
#86978=ADVANCED_FACE ( 'NONE', ( #88530 ), #33562, .F. ) ;
#87063=MECHANICAL_DESIGN_GEOMETRIC_PRESENTATION_REPRESENTATION('',(#26576),#70405);
#87260=VERTEX_POINT ( 'NONE', #25988 ) ;
#87369=EDGE_CURVE ( 'NONE', #32191, #86290, #13224, .T. ) ;
#87716=ORIENTED_EDGE ( 'NONE', *, *, #92091, .F. ) ;
#87766=AXIS2_PLACEMENT_3D ( 'NONE', #3055, #39473, #61312 ) ;
#87773=EDGE_CURVE ( 'NONE', #91222, #43507, #19749, .T. ) ;
#87852=FACE_OUTER_BOUND ( 'NONE', #90554, .T. ) ;
#88063=ORIENTED_EDGE ( 'NONE', *, *, #26993, .F. ) ;
#88219=EDGE_LOOP ( 'NONE', ( #52109, #88996, #442, #40316 ) ) ;
#88344=ORIENTED_EDGE ( 'NONE', *, *, #92638, .T. ) ;
#88428=DIRECTION ( 'NONE',  ( -0.000000000000000000, 1.000000000000000000, -0.000000000000000000 ) ) ;
#88530=FACE_OUTER_BOUND ( 'NONE', #15625, .T. ) ;
#88600=VECTOR ( 'NONE', #68059, 1000.000000000000000 ) ;
#88840=EDGE_CURVE ( 'NONE', #92631, #9616, #64844, .T. ) ;
#88842=DIRECTION ( 'NONE',  ( -1.000000000000000000, -0.000000000000000000, -0.000000000000000000 ) ) ;
#88943=EDGE_CURVE ( 'NONE', #32344, #59329, #1792, .T. ) ;
#88996=ORIENTED_EDGE ( 'NONE', *, *, #68227, .F. ) ;
#89023=DIRECTION ( 'NONE',  ( 0.000000000000000000, 0.9681751575201845705, -0.2502735790305594121 ) ) ;
#89059=CYLINDRICAL_SURFACE ( 'NONE', #86631, 28.04691768583012035 ) ;
#89272=CARTESIAN_POINT ( 'NONE',  ( 113.5000000000000568, -296.0521521680024080, -537.7509286889328450 ) ) ;
#89336=CARTESIAN_POINT ( 'NONE',  ( 113.5000000000000568, -298.0521521680024080, -540.3336712212508246 ) ) ;
#89467=EDGE_LOOP ( 'NONE', ( #2307, #42924, #6796, #76758 ) ) ;
#89695=EDGE_CURVE ( 'NONE', #42343, #87260, #70339, .T. ) ;
#89762=DIRECTION ( 'NONE',  ( 0.000000000000000000, 0.000000000000000000, 1.000000000000000000 ) ) ;
#89804=FACE_OUTER_BOUND ( 'NONE', #38014, .T. ) ;
#90276=DIRECTION ( 'NONE',  ( -0.000000000000000000, 1.000000000000000000, -0.000000000000000000 ) ) ;
#90366=ADVANCED_FACE ( 'NONE', ( #87852, #65205 ), #1238, .T. ) ;
#90372=CARTESIAN_POINT ( 'NONE',  ( 113.5000000000000568, -298.0521521680024080, -540.3336712212508246 ) ) ;
#90554=EDGE_LOOP ( 'NONE', ( #87716, #86799, #88063, #19828, #42462, #74256 ) ) ;
#90555=CYLINDRICAL_SURFACE ( 'NONE', #50140, 4.000000000000003553 ) ;
#90665=LINE ( 'NONE', #25825, #72405 ) ;
#90715=DIRECTION ( 'NONE',  ( -0.000000000000000000, 1.000000000000000000, -0.000000000000000000 ) ) ;
#90800=DIRECTION ( 'NONE',  ( 0.000000000000000000, 0.000000000000000000, 1.000000000000000000 ) ) ;
#90881=CARTESIAN_POINT ( 'NONE',  ( 85.55100297371598117, -298.0521521680024080, -417.1172536214571096 ) ) ;
#90959=CARTESIAN_POINT ( 'NONE',  ( 0.000000000000000000, 0.000000000000000000, 0.000000000000000000 ) ) ;
#91058=AXIS2_PLACEMENT_3D ( 'NONE', #25499, #82789, #90800 ) ;
#91112=CARTESIAN_POINT ( 'NONE',  ( 85.55100297371609486, -373.0521521680024648, -521.1711561948568487 ) ) ;
#91220=MANIFOLD_SOLID_BREP ( 'Cut-Extrude10', #29514 ) ;
#91222=VERTEX_POINT ( 'NONE', #13690 ) ;
#91285=CARTESIAN_POINT ( 'NONE',  ( -83.63170945779074827, -373.0521521680024648, -521.1711561948568487 ) ) ;
#91438=( GEOMETRIC_REPRESENTATION_CONTEXT ( 3 ) GLOBAL_UNCERTAINTY_ASSIGNED_CONTEXT ( ( #70329 ) ) GLOBAL_UNIT_ASSIGNED_CONTEXT ( ( #7172, #77265, #63088 ) ) REPRESENTATION_CONTEXT ( 'NONE', 'WORKASPACE' ) );
#91514=DIRECTION ( 'NONE',  ( -0.000000000000000000, 1.000000000000000000, -0.000000000000000000 ) ) ;
#91516=DIRECTION ( 'NONE',  ( 0.000000000000000000, 0.000000000000000000, -1.000000000000000000 ) ) ;
#91691=ORIENTED_EDGE ( 'NONE', *, *, #47636, .F. ) ;
#91946=ORIENTED_EDGE ( 'NONE', *, *, #34351, .F. ) ;
#92091=EDGE_CURVE ( 'NONE', #87260, #26725, #65769, .T. ) ;
#92152=CARTESIAN_POINT ( 'NONE',  ( 113.5000000000000568, -218.8335761803644743, -447.4016117689005796 ) ) ;
#92178=AXIS2_PLACEMENT_3D ( 'NONE', #77918, #36209, #65128 ) ;
#92351=DIRECTION ( 'NONE',  ( -0.000000000000000000, 1.000000000000000000, 0.000000000000000000 ) ) ;
#92435=CYLINDRICAL_SURFACE ( 'NONE', #4990, 4.000000000000003553 ) ;
#92547=CARTESIAN_POINT ( 'NONE',  ( 113.5000000000000568, -218.8335761803644743, -447.4016117689005796 ) ) ;
#92559=PLANE ( 'NONE',  #92793 ) ;
#92612=EDGE_CURVE ( 'NONE', #47975, #33034, #54768, .T. ) ;
#92631=VERTEX_POINT ( 'NONE', #25427 ) ;
#92638=EDGE_CURVE ( 'NONE', #24966, #36396, #11690, .T. ) ;
#92713=AXIS2_PLACEMENT_3D ( 'NONE', #7537, #71495, #49234 ) ;
#92793=AXIS2_PLACEMENT_3D ( 'NONE', #57089, #71285, #64676 ) ;
#93145=FACE_BOUND ( 'NONE', #44508, .T. ) ;
#93231=VERTEX_POINT ( 'NONE', #62854 ) ;
#93458=EDGE_CURVE ( 'NONE', #59451, #42812, #46038, .T. ) ;
#93474=AXIS2_PLACEMENT_3D ( 'NONE', #84536, #48552, #20637 ) ;
#93574=CARTESIAN_POINT ( 'NONE',  ( 113.5000000000000568, -298.0521521680024080, -540.3336712212508246 ) ) ;
#93668=CARTESIAN_POINT ( 'NONE',  ( 85.55100297371598117, -298.0521521680024080, -421.1172536214571096 ) ) ;
#93739=COLOUR_RGB('Sky Blue',0.24,0.69,0.87);
#93740=FILL_AREA_STYLE_COLOUR('',#93739);
#93741=FILL_AREA_STYLE('',(#93740));
#93742=SURFACE_STYLE_FILL_AREA(#93741);
#93743=SURFACE_SIDE_STYLE('',(#93742));
#93744=SURFACE_STYLE_USAGE(.BOTH.,#93743);
#93745=PRESENTATION_STYLE_ASSIGNMENT((#93744));
ENDSEC;
END-ISO-10303-21;
